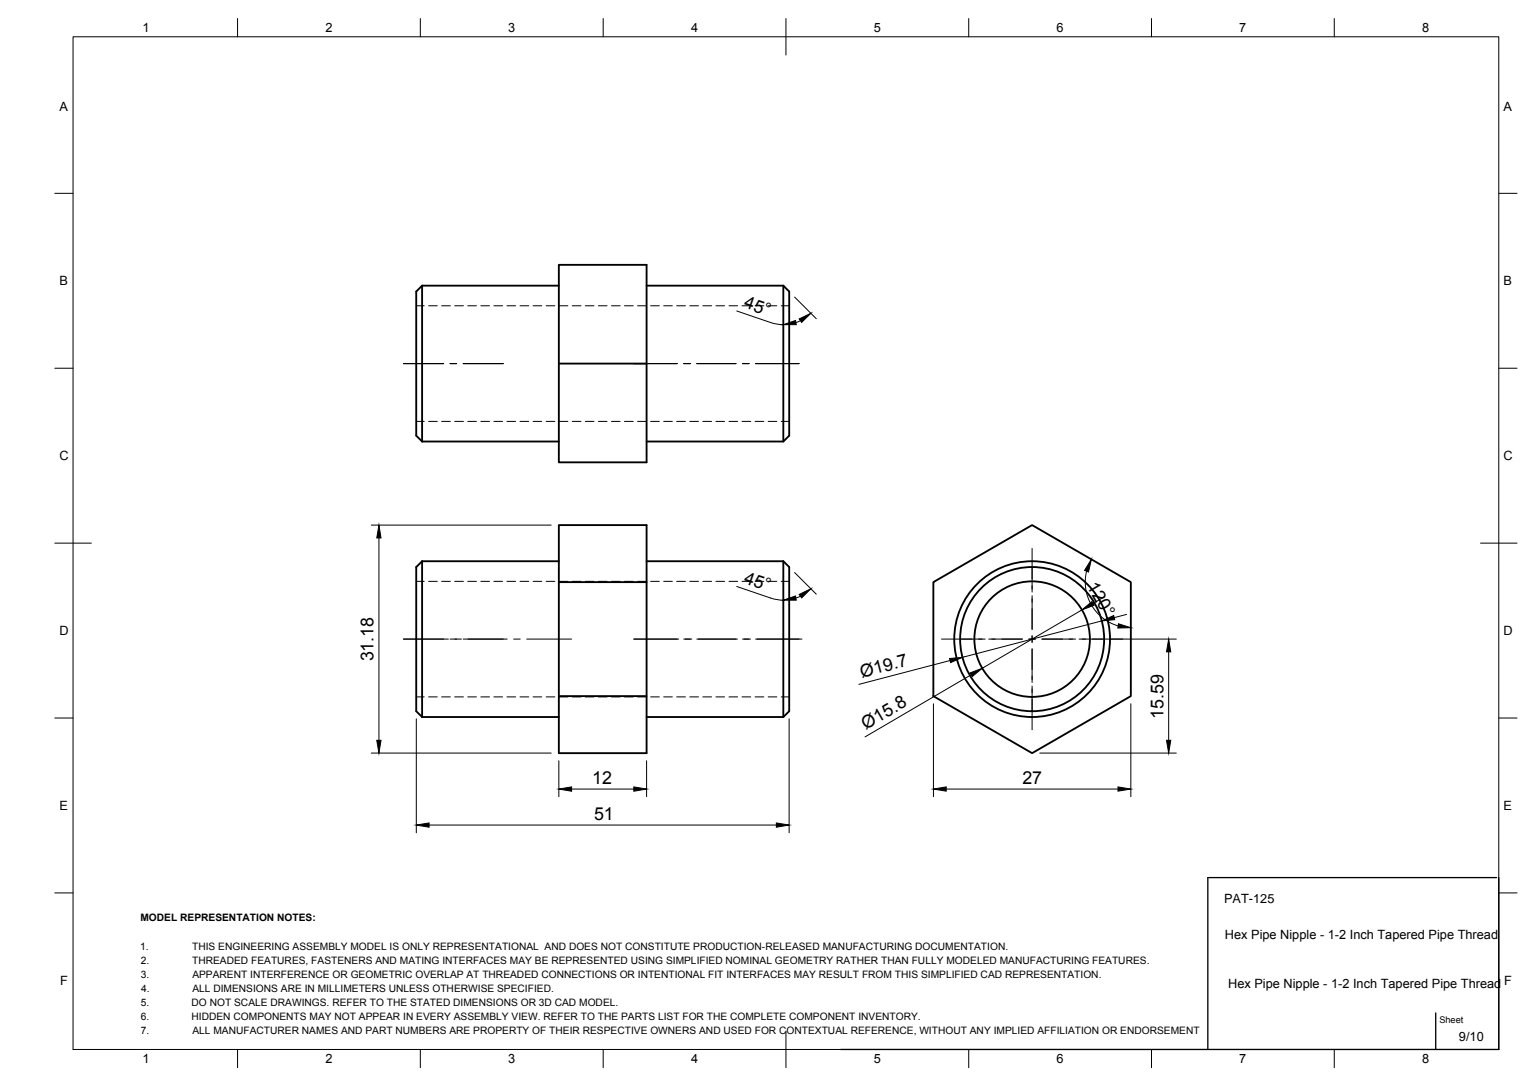
ISO-10303-21;
HEADER;
/* Generated by software containing ST-Developer
 * from STEP Tools, Inc. (www.steptools.com) 
 */

FILE_DESCRIPTION(
/* description */ ('Y-strainer with drain'),
/* implementation_level */ '2;1');

FILE_NAME(
/* name */ 'Hex Pipe Nipple - 1-2 Inch Tapered Pipe Thread.step',
/* time_stamp */ '2026-10-28T00:41:55-07:00',
/* author */ (''),
/* organization */ (''),
/* preprocessor_version */ 'ST-DEVELOPER v20.2',
/* originating_system */ 'Autodesk Translation Framework v15.17.0.0',
/* authorisation */ '');

FILE_SCHEMA (('AUTOMOTIVE_DESIGN { 1 0 10303 214 3 1 1 }'));
ENDSEC;

DATA;
#10=MECHANICAL_DESIGN_GEOMETRIC_PRESENTATION_REPRESENTATION('',(#100),#8864);
#72=CONICAL_SURFACE('',#3736,1.025,0.785398163397448);
#73=CONICAL_SURFACE('',#3739,1.025,0.785398163397448);
#82=SHAPE_REPRESENTATION_RELATIONSHIP('SRR','None',#8914,#91);
#91=ADVANCED_BREP_SHAPE_REPRESENTATION('',(#108),#8862);
#100=STYLED_ITEM('',(#9019),#108);
#108=MANIFOLD_SOLID_BREP('Body1',#3391);
#451=FACE_BOUND('',#932,.T.);
#452=FACE_BOUND('',#934,.T.);
#453=FACE_BOUND('',#943,.T.);
#454=FACE_BOUND('',#948,.T.);
#501=PLANE('',#3721);
#502=PLANE('',#3723);
#503=PLANE('',#3725);
#504=PLANE('',#3726);
#505=PLANE('',#3727);
#506=PLANE('',#3728);
#507=PLANE('',#3729);
#508=PLANE('',#3730);
#509=PLANE('',#3733);
#510=PLANE('',#3741);
#647=FACE_OUTER_BOUND('',#931,.T.);
#648=FACE_OUTER_BOUND('',#933,.T.);
#649=FACE_OUTER_BOUND('',#935,.T.);
#650=FACE_OUTER_BOUND('',#936,.T.);
#651=FACE_OUTER_BOUND('',#937,.T.);
#652=FACE_OUTER_BOUND('',#938,.T.);
#653=FACE_OUTER_BOUND('',#939,.T.);
#654=FACE_OUTER_BOUND('',#940,.T.);
#655=FACE_OUTER_BOUND('',#941,.T.);
#656=FACE_OUTER_BOUND('',#942,.T.);
#657=FACE_OUTER_BOUND('',#944,.T.);
#658=FACE_OUTER_BOUND('',#945,.T.);
#659=FACE_OUTER_BOUND('',#946,.T.);
#660=FACE_OUTER_BOUND('',#947,.T.);
#661=FACE_OUTER_BOUND('',#949,.T.);
#931=EDGE_LOOP('',(#3036,#3037,#3038,#3039,#3040,#3041));
#932=EDGE_LOOP('',(#3042));
#933=EDGE_LOOP('',(#3043,#3044,#3045,#3046,#3047,#3048));
#934=EDGE_LOOP('',(#3049));
#935=EDGE_LOOP('',(#3050,#3051,#3052,#3053));
#936=EDGE_LOOP('',(#3054,#3055,#3056,#3057));
#937=EDGE_LOOP('',(#3058,#3059,#3060,#3061));
#938=EDGE_LOOP('',(#3062,#3063,#3064,#3065));
#939=EDGE_LOOP('',(#3066,#3067,#3068,#3069));
#940=EDGE_LOOP('',(#3070,#3071,#3072,#3073));
#941=EDGE_LOOP('',(#3074,#3075,#3076,#3077));
#942=EDGE_LOOP('',(#3078));
#943=EDGE_LOOP('',(#3079));
#944=EDGE_LOOP('',(#3080,#3081,#3082,#3083));
#945=EDGE_LOOP('',(#3084,#3085,#3086,#3087));
#946=EDGE_LOOP('',(#3088,#3089,#3090,#3091));
#947=EDGE_LOOP('',(#3092));
#948=EDGE_LOOP('',(#3093));
#949=EDGE_LOOP('',(#3094,#3095,#3096,#3097));
#1082=LINE('',#8718,#1245);
#1083=LINE('',#8720,#1246);
#1084=LINE('',#8722,#1247);
#1085=LINE('',#8724,#1248);
#1086=LINE('',#8726,#1249);
#1087=LINE('',#8727,#1250);
#1088=LINE('',#8733,#1251);
#1089=LINE('',#8735,#1252);
#1090=LINE('',#8737,#1253);
#1091=LINE('',#8739,#1254);
#1092=LINE('',#8741,#1255);
#1093=LINE('',#8742,#1256);
#1094=LINE('',#8746,#1257);
#1095=LINE('',#8747,#1258);
#1096=LINE('',#8749,#1259);
#1097=LINE('',#8751,#1260);
#1098=LINE('',#8753,#1261);
#1099=LINE('',#8755,#1262);
#1100=LINE('',#8759,#1263);
#1101=LINE('',#8767,#1264);
#1102=LINE('',#8771,#1265);
#1103=LINE('',#8775,#1266);
#1104=LINE('',#8780,#1267);
#1245=VECTOR('',#4350,1.);
#1246=VECTOR('',#4351,1.);
#1247=VECTOR('',#4352,1.);
#1248=VECTOR('',#4353,1.);
#1249=VECTOR('',#4354,1.);
#1250=VECTOR('',#4355,1.);
#1251=VECTOR('',#4360,1.);
#1252=VECTOR('',#4361,1.);
#1253=VECTOR('',#4362,1.);
#1254=VECTOR('',#4363,1.);
#1255=VECTOR('',#4364,1.);
#1256=VECTOR('',#4365,1.);
#1257=VECTOR('',#4370,1.);
#1258=VECTOR('',#4371,1.);
#1259=VECTOR('',#4374,1.);
#1260=VECTOR('',#4377,1.);
#1261=VECTOR('',#4380,1.);
#1262=VECTOR('',#4383,1.);
#1263=VECTOR('',#4388,1.065);
#1264=VECTOR('',#4399,1.025);
#1265=VECTOR('',#4404,1.065);
#1266=VECTOR('',#4409,1.025);
#1267=VECTOR('',#4416,0.79);
#1369=CIRCLE('',#3722,1.065);
#1370=CIRCLE('',#3724,1.065);
#1371=CIRCLE('',#3732,1.065);
#1372=CIRCLE('',#3734,0.985);
#1373=CIRCLE('',#3735,0.79);
#1374=CIRCLE('',#3738,1.065);
#1375=CIRCLE('',#3740,0.985);
#1376=CIRCLE('',#3742,0.79);
#1687=VERTEX_POINT('',#8716);
#1688=VERTEX_POINT('',#8717);
#1689=VERTEX_POINT('',#8719);
#1690=VERTEX_POINT('',#8721);
#1691=VERTEX_POINT('',#8723);
#1692=VERTEX_POINT('',#8725);
#1693=VERTEX_POINT('',#8728);
#1694=VERTEX_POINT('',#8731);
#1695=VERTEX_POINT('',#8732);
#1696=VERTEX_POINT('',#8734);
#1697=VERTEX_POINT('',#8736);
#1698=VERTEX_POINT('',#8738);
#1699=VERTEX_POINT('',#8740);
#1700=VERTEX_POINT('',#8743);
#1701=VERTEX_POINT('',#8758);
#1702=VERTEX_POINT('',#8762);
#1703=VERTEX_POINT('',#8764);
#1704=VERTEX_POINT('',#8769);
#1705=VERTEX_POINT('',#8773);
#1706=VERTEX_POINT('',#8777);
#2142=EDGE_CURVE('',#1687,#1688,#1082,.T.);
#2143=EDGE_CURVE('',#1688,#1689,#1083,.T.);
#2144=EDGE_CURVE('',#1689,#1690,#1084,.T.);
#2145=EDGE_CURVE('',#1690,#1691,#1085,.T.);
#2146=EDGE_CURVE('',#1691,#1692,#1086,.T.);
#2147=EDGE_CURVE('',#1692,#1687,#1087,.T.);
#2148=EDGE_CURVE('',#1693,#1693,#1369,.T.);
#2149=EDGE_CURVE('',#1694,#1695,#1088,.T.);
#2150=EDGE_CURVE('',#1695,#1696,#1089,.T.);
#2151=EDGE_CURVE('',#1696,#1697,#1090,.T.);
#2152=EDGE_CURVE('',#1697,#1698,#1091,.T.);
#2153=EDGE_CURVE('',#1698,#1699,#1092,.T.);
#2154=EDGE_CURVE('',#1699,#1694,#1093,.T.);
#2155=EDGE_CURVE('',#1700,#1700,#1370,.T.);
#2156=EDGE_CURVE('',#1694,#1688,#1094,.T.);
#2157=EDGE_CURVE('',#1689,#1699,#1095,.T.);
#2158=EDGE_CURVE('',#1690,#1698,#1096,.T.);
#2159=EDGE_CURVE('',#1691,#1697,#1097,.T.);
#2160=EDGE_CURVE('',#1692,#1696,#1098,.T.);
#2161=EDGE_CURVE('',#1687,#1695,#1099,.T.);
#2162=EDGE_CURVE('',#1700,#1701,#1100,.T.);
#2163=EDGE_CURVE('',#1701,#1701,#1371,.T.);
#2164=EDGE_CURVE('',#1702,#1702,#1372,.T.);
#2165=EDGE_CURVE('',#1703,#1703,#1373,.T.);
#2166=EDGE_CURVE('',#1701,#1702,#1101,.T.);
#2167=EDGE_CURVE('',#1704,#1704,#1374,.T.);
#2168=EDGE_CURVE('',#1704,#1693,#1102,.T.);
#2169=EDGE_CURVE('',#1705,#1705,#1375,.T.);
#2170=EDGE_CURVE('',#1705,#1704,#1103,.T.);
#2171=EDGE_CURVE('',#1706,#1706,#1376,.T.);
#2172=EDGE_CURVE('',#1706,#1703,#1104,.T.);
#3036=ORIENTED_EDGE('',*,*,#2142,.T.);
#3037=ORIENTED_EDGE('',*,*,#2143,.T.);
#3038=ORIENTED_EDGE('',*,*,#2144,.T.);
#3039=ORIENTED_EDGE('',*,*,#2145,.T.);
#3040=ORIENTED_EDGE('',*,*,#2146,.T.);
#3041=ORIENTED_EDGE('',*,*,#2147,.T.);
#3042=ORIENTED_EDGE('',*,*,#2148,.F.);
#3043=ORIENTED_EDGE('',*,*,#2149,.T.);
#3044=ORIENTED_EDGE('',*,*,#2150,.T.);
#3045=ORIENTED_EDGE('',*,*,#2151,.T.);
#3046=ORIENTED_EDGE('',*,*,#2152,.T.);
#3047=ORIENTED_EDGE('',*,*,#2153,.T.);
#3048=ORIENTED_EDGE('',*,*,#2154,.T.);
#3049=ORIENTED_EDGE('',*,*,#2155,.F.);
#3050=ORIENTED_EDGE('',*,*,#2156,.F.);
#3051=ORIENTED_EDGE('',*,*,#2154,.F.);
#3052=ORIENTED_EDGE('',*,*,#2157,.F.);
#3053=ORIENTED_EDGE('',*,*,#2143,.F.);
#3054=ORIENTED_EDGE('',*,*,#2157,.T.);
#3055=ORIENTED_EDGE('',*,*,#2153,.F.);
#3056=ORIENTED_EDGE('',*,*,#2158,.F.);
#3057=ORIENTED_EDGE('',*,*,#2144,.F.);
#3058=ORIENTED_EDGE('',*,*,#2158,.T.);
#3059=ORIENTED_EDGE('',*,*,#2152,.F.);
#3060=ORIENTED_EDGE('',*,*,#2159,.F.);
#3061=ORIENTED_EDGE('',*,*,#2145,.F.);
#3062=ORIENTED_EDGE('',*,*,#2159,.T.);
#3063=ORIENTED_EDGE('',*,*,#2151,.F.);
#3064=ORIENTED_EDGE('',*,*,#2160,.F.);
#3065=ORIENTED_EDGE('',*,*,#2146,.F.);
#3066=ORIENTED_EDGE('',*,*,#2160,.T.);
#3067=ORIENTED_EDGE('',*,*,#2150,.F.);
#3068=ORIENTED_EDGE('',*,*,#2161,.F.);
#3069=ORIENTED_EDGE('',*,*,#2147,.F.);
#3070=ORIENTED_EDGE('',*,*,#2161,.T.);
#3071=ORIENTED_EDGE('',*,*,#2149,.F.);
#3072=ORIENTED_EDGE('',*,*,#2156,.T.);
#3073=ORIENTED_EDGE('',*,*,#2142,.F.);
#3074=ORIENTED_EDGE('',*,*,#2155,.T.);
#3075=ORIENTED_EDGE('',*,*,#2162,.T.);
#3076=ORIENTED_EDGE('',*,*,#2163,.T.);
#3077=ORIENTED_EDGE('',*,*,#2162,.F.);
#3078=ORIENTED_EDGE('',*,*,#2164,.F.);
#3079=ORIENTED_EDGE('',*,*,#2165,.T.);
#3080=ORIENTED_EDGE('',*,*,#2163,.F.);
#3081=ORIENTED_EDGE('',*,*,#2166,.T.);
#3082=ORIENTED_EDGE('',*,*,#2164,.T.);
#3083=ORIENTED_EDGE('',*,*,#2166,.F.);
#3084=ORIENTED_EDGE('',*,*,#2167,.F.);
#3085=ORIENTED_EDGE('',*,*,#2168,.T.);
#3086=ORIENTED_EDGE('',*,*,#2148,.T.);
#3087=ORIENTED_EDGE('',*,*,#2168,.F.);
#3088=ORIENTED_EDGE('',*,*,#2169,.F.);
#3089=ORIENTED_EDGE('',*,*,#2170,.T.);
#3090=ORIENTED_EDGE('',*,*,#2167,.T.);
#3091=ORIENTED_EDGE('',*,*,#2170,.F.);
#3092=ORIENTED_EDGE('',*,*,#2169,.T.);
#3093=ORIENTED_EDGE('',*,*,#2171,.F.);
#3094=ORIENTED_EDGE('',*,*,#2171,.T.);
#3095=ORIENTED_EDGE('',*,*,#2172,.T.);
#3096=ORIENTED_EDGE('',*,*,#2165,.F.);
#3097=ORIENTED_EDGE('',*,*,#2172,.F.);
#3227=CYLINDRICAL_SURFACE('',#3731,1.065);
#3228=CYLINDRICAL_SURFACE('',#3737,1.065);
#3229=CYLINDRICAL_SURFACE('',#3743,0.79);
#3358=ADVANCED_FACE('',(#647,#451),#501,.F.);
#3359=ADVANCED_FACE('',(#648,#452),#502,.T.);
#3360=ADVANCED_FACE('',(#649),#503,.T.);
#3361=ADVANCED_FACE('',(#650),#504,.T.);
#3362=ADVANCED_FACE('',(#651),#505,.T.);
#3363=ADVANCED_FACE('',(#652),#506,.T.);
#3364=ADVANCED_FACE('',(#653),#507,.T.);
#3365=ADVANCED_FACE('',(#654),#508,.T.);
#3366=ADVANCED_FACE('',(#655),#3227,.T.);
#3367=ADVANCED_FACE('',(#656,#453),#509,.T.);
#3368=ADVANCED_FACE('',(#657),#72,.T.);
#3369=ADVANCED_FACE('',(#658),#3228,.T.);
#3370=ADVANCED_FACE('',(#659),#73,.T.);
#3371=ADVANCED_FACE('',(#660,#454),#510,.T.);
#3372=ADVANCED_FACE('',(#661),#3229,.F.);
#3391=CLOSED_SHELL('',(#3358,#3359,#3360,#3361,#3362,#3363,#3364,#3365,
#3366,#3367,#3368,#3369,#3370,#3371,#3372));
#3720=AXIS2_PLACEMENT_3D('',#8714,#4346,#4347);
#3721=AXIS2_PLACEMENT_3D('',#8715,#4348,#4349);
#3722=AXIS2_PLACEMENT_3D('',#8729,#4356,#4357);
#3723=AXIS2_PLACEMENT_3D('',#8730,#4358,#4359);
#3724=AXIS2_PLACEMENT_3D('',#8744,#4366,#4367);
#3725=AXIS2_PLACEMENT_3D('',#8745,#4368,#4369);
#3726=AXIS2_PLACEMENT_3D('',#8748,#4372,#4373);
#3727=AXIS2_PLACEMENT_3D('',#8750,#4375,#4376);
#3728=AXIS2_PLACEMENT_3D('',#8752,#4378,#4379);
#3729=AXIS2_PLACEMENT_3D('',#8754,#4381,#4382);
#3730=AXIS2_PLACEMENT_3D('',#8756,#4384,#4385);
#3731=AXIS2_PLACEMENT_3D('',#8757,#4386,#4387);
#3732=AXIS2_PLACEMENT_3D('',#8760,#4389,#4390);
#3733=AXIS2_PLACEMENT_3D('',#8761,#4391,#4392);
#3734=AXIS2_PLACEMENT_3D('',#8763,#4393,#4394);
#3735=AXIS2_PLACEMENT_3D('',#8765,#4395,#4396);
#3736=AXIS2_PLACEMENT_3D('',#8766,#4397,#4398);
#3737=AXIS2_PLACEMENT_3D('',#8768,#4400,#4401);
#3738=AXIS2_PLACEMENT_3D('',#8770,#4402,#4403);
#3739=AXIS2_PLACEMENT_3D('',#8772,#4405,#4406);
#3740=AXIS2_PLACEMENT_3D('',#8774,#4407,#4408);
#3741=AXIS2_PLACEMENT_3D('',#8776,#4410,#4411);
#3742=AXIS2_PLACEMENT_3D('',#8778,#4412,#4413);
#3743=AXIS2_PLACEMENT_3D('',#8779,#4414,#4415);
#4346=DIRECTION('axis',(0.,0.,1.));
#4347=DIRECTION('refdir',(1.,0.,0.));
#4348=DIRECTION('center_axis',(0.,1.,0.));
#4349=DIRECTION('ref_axis',(1.,0.,0.));
#4350=DIRECTION('',(-0.5,0.,0.866025403784439));
#4351=DIRECTION('',(-1.,0.,-2.84883360945713E-16));
#4352=DIRECTION('',(-0.5,0.,-0.866025403784439));
#4353=DIRECTION('',(0.5,0.,-0.866025403784439));
#4354=DIRECTION('',(1.,0.,0.));
#4355=DIRECTION('',(0.5,0.,0.866025403784439));
#4356=DIRECTION('center_axis',(0.,-1.,0.));
#4357=DIRECTION('ref_axis',(1.,0.,0.));
#4358=DIRECTION('center_axis',(0.,1.,0.));
#4359=DIRECTION('ref_axis',(1.,0.,0.));
#4360=DIRECTION('',(0.5,0.,-0.866025403784439));
#4361=DIRECTION('',(-0.5,0.,-0.866025403784439));
#4362=DIRECTION('',(-1.,0.,0.));
#4363=DIRECTION('',(-0.5,0.,0.866025403784439));
#4364=DIRECTION('',(0.5,0.,0.866025403784439));
#4365=DIRECTION('',(1.,0.,2.84883360945713E-16));
#4366=DIRECTION('center_axis',(0.,1.,0.));
#4367=DIRECTION('ref_axis',(1.,0.,0.));
#4368=DIRECTION('center_axis',(-2.84883360945713E-16,0.,1.));
#4369=DIRECTION('ref_axis',(1.,0.,2.84883360945713E-16));
#4370=DIRECTION('',(0.,-1.,0.));
#4371=DIRECTION('',(0.,1.,0.));
#4372=DIRECTION('center_axis',(-0.866025403784439,0.,0.5));
#4373=DIRECTION('ref_axis',(0.5,0.,0.866025403784439));
#4374=DIRECTION('',(0.,1.,0.));
#4375=DIRECTION('center_axis',(-0.866025403784439,0.,-0.5));
#4376=DIRECTION('ref_axis',(-0.5,0.,0.866025403784439));
#4377=DIRECTION('',(0.,1.,0.));
#4378=DIRECTION('center_axis',(0.,0.,-1.));
#4379=DIRECTION('ref_axis',(-1.,0.,0.));
#4380=DIRECTION('',(0.,1.,0.));
#4381=DIRECTION('center_axis',(0.866025403784439,0.,-0.5));
#4382=DIRECTION('ref_axis',(-0.5,0.,-0.866025403784439));
#4383=DIRECTION('',(0.,1.,0.));
#4384=DIRECTION('center_axis',(0.866025403784439,0.,0.5));
#4385=DIRECTION('ref_axis',(0.5,0.,-0.866025403784439));
#4386=DIRECTION('center_axis',(0.,-1.,0.));
#4387=DIRECTION('ref_axis',(1.,0.,0.));
#4388=DIRECTION('',(0.,1.,0.));
#4389=DIRECTION('center_axis',(0.,-1.,0.));
#4390=DIRECTION('ref_axis',(1.,0.,0.));
#4391=DIRECTION('center_axis',(0.,1.,0.));
#4392=DIRECTION('ref_axis',(0.,0.,1.));
#4393=DIRECTION('center_axis',(0.,-1.,0.));
#4394=DIRECTION('ref_axis',(1.,0.,0.));
#4395=DIRECTION('center_axis',(0.,-1.,0.));
#4396=DIRECTION('ref_axis',(1.,0.,0.));
#4397=DIRECTION('center_axis',(0.,-1.,0.));
#4398=DIRECTION('ref_axis',(1.,0.,0.));
#4399=DIRECTION('',(0.707106781186547,0.707106781186548,8.65956056235493E-17));
#4400=DIRECTION('center_axis',(0.,-1.,0.));
#4401=DIRECTION('ref_axis',(1.,0.,0.));
#4402=DIRECTION('center_axis',(0.,-1.,0.));
#4403=DIRECTION('ref_axis',(1.,0.,0.));
#4404=DIRECTION('',(0.,1.,0.));
#4405=DIRECTION('center_axis',(0.,1.,0.));
#4406=DIRECTION('ref_axis',(1.,0.,0.));
#4407=DIRECTION('center_axis',(0.,-1.,0.));
#4408=DIRECTION('ref_axis',(1.,0.,0.));
#4409=DIRECTION('',(-0.707106781186547,0.707106781186548,-8.65956056235493E-17));
#4410=DIRECTION('center_axis',(0.,-1.,0.));
#4411=DIRECTION('ref_axis',(0.,0.,-1.));
#4412=DIRECTION('center_axis',(0.,-1.,0.));
#4413=DIRECTION('ref_axis',(1.,0.,0.));
#4414=DIRECTION('center_axis',(0.,-1.,0.));
#4415=DIRECTION('ref_axis',(1.,0.,0.));
#4416=DIRECTION('',(0.,1.,0.));
#8714=CARTESIAN_POINT('',(0.,0.,0.));
#8715=CARTESIAN_POINT('Origin',(0.,-0.6,0.));
#8716=CARTESIAN_POINT('',(1.55884572681199,-0.6,0.));
#8717=CARTESIAN_POINT('',(0.779422863405995,-0.6,1.35));
#8718=CARTESIAN_POINT('',(0.779422863405995,-0.6,1.35));
#8719=CARTESIAN_POINT('',(-0.779422863405996,-0.6,1.35));
#8720=CARTESIAN_POINT('',(-0.779422863405996,-0.6,1.35));
#8721=CARTESIAN_POINT('',(-1.55884572681199,-0.6,-1.90903542970483E-16));
#8722=CARTESIAN_POINT('',(-1.55884572681199,-0.6,-1.90903542970483E-16));
#8723=CARTESIAN_POINT('',(-0.779422863405995,-0.6,-1.35));
#8724=CARTESIAN_POINT('',(-0.779422863405995,-0.6,-1.35));
#8725=CARTESIAN_POINT('',(0.779422863405995,-0.6,-1.35));
#8726=CARTESIAN_POINT('',(0.779422863405995,-0.6,-1.35));
#8727=CARTESIAN_POINT('',(1.55884572681199,-0.6,0.));
#8728=CARTESIAN_POINT('',(-1.065,-0.6,-1.30424884109193E-16));
#8729=CARTESIAN_POINT('Origin',(0.,-0.6,0.));
#8730=CARTESIAN_POINT('Origin',(0.,0.6,0.));
#8731=CARTESIAN_POINT('',(0.779422863405995,0.6,1.35));
#8732=CARTESIAN_POINT('',(1.55884572681199,0.6,0.));
#8733=CARTESIAN_POINT('',(0.779422863405995,0.6,1.35));
#8734=CARTESIAN_POINT('',(0.779422863405995,0.6,-1.35));
#8735=CARTESIAN_POINT('',(1.55884572681199,0.6,0.));
#8736=CARTESIAN_POINT('',(-0.779422863405995,0.6,-1.35));
#8737=CARTESIAN_POINT('',(0.779422863405995,0.6,-1.35));
#8738=CARTESIAN_POINT('',(-1.55884572681199,0.6,-1.90903542970483E-16));
#8739=CARTESIAN_POINT('',(-0.779422863405995,0.6,-1.35));
#8740=CARTESIAN_POINT('',(-0.779422863405996,0.6,1.35));
#8741=CARTESIAN_POINT('',(-1.55884572681199,0.6,-1.90903542970483E-16));
#8742=CARTESIAN_POINT('',(-0.779422863405996,0.6,1.35));
#8743=CARTESIAN_POINT('',(-1.065,0.6,1.30424884109193E-16));
#8744=CARTESIAN_POINT('Origin',(0.,0.6,0.));
#8745=CARTESIAN_POINT('Origin',(-0.779422863405996,0.,1.35));
#8746=CARTESIAN_POINT('',(0.779422863405995,0.,1.35));
#8747=CARTESIAN_POINT('',(-0.779422863405996,0.,1.35));
#8748=CARTESIAN_POINT('Origin',(-1.55884572681199,0.,-1.90903542970483E-16));
#8749=CARTESIAN_POINT('',(-1.55884572681199,0.,-1.90903542970483E-16));
#8750=CARTESIAN_POINT('Origin',(-0.779422863405995,0.,-1.35));
#8751=CARTESIAN_POINT('',(-0.779422863405995,0.,-1.35));
#8752=CARTESIAN_POINT('Origin',(0.779422863405995,0.,-1.35));
#8753=CARTESIAN_POINT('',(0.779422863405995,0.,-1.35));
#8754=CARTESIAN_POINT('Origin',(1.55884572681199,0.,0.));
#8755=CARTESIAN_POINT('',(1.55884572681199,0.,0.));
#8756=CARTESIAN_POINT('Origin',(0.779422863405995,0.,1.35));
#8757=CARTESIAN_POINT('Origin',(0.,0.,0.));
#8758=CARTESIAN_POINT('',(-1.065,2.47,-1.30424884109193E-16));
#8759=CARTESIAN_POINT('',(-1.065,0.,-1.30424884109193E-16));
#8760=CARTESIAN_POINT('Origin',(0.,2.47,0.));
#8761=CARTESIAN_POINT('Origin',(0.985,2.55,0.));
#8762=CARTESIAN_POINT('',(-0.985,2.55,-1.20627709716014E-16));
#8763=CARTESIAN_POINT('Origin',(0.,2.55,0.));
#8764=CARTESIAN_POINT('',(-0.79,2.55,-9.67470971326409E-17));
#8765=CARTESIAN_POINT('Origin',(0.,2.55,0.));
#8766=CARTESIAN_POINT('Origin',(0.,2.51,0.));
#8767=CARTESIAN_POINT('',(-1.025,2.51,-1.25526296912604E-16));
#8768=CARTESIAN_POINT('Origin',(0.,0.,0.));
#8769=CARTESIAN_POINT('',(-1.065,-2.47,-1.30424884109193E-16));
#8770=CARTESIAN_POINT('Origin',(0.,-2.47,0.));
#8771=CARTESIAN_POINT('',(-1.065,0.,-1.30424884109193E-16));
#8772=CARTESIAN_POINT('Origin',(0.,-2.51,0.));
#8773=CARTESIAN_POINT('',(-0.985,-2.55,-1.20627709716014E-16));
#8774=CARTESIAN_POINT('Origin',(0.,-2.55,0.));
#8775=CARTESIAN_POINT('',(-1.025,-2.51,-1.25526296912604E-16));
#8776=CARTESIAN_POINT('Origin',(0.79,-2.55,0.));
#8777=CARTESIAN_POINT('',(-0.79,-2.55,-9.67470971326409E-17));
#8778=CARTESIAN_POINT('Origin',(0.,-2.55,0.));
#8779=CARTESIAN_POINT('Origin',(0.,0.,0.));
#8780=CARTESIAN_POINT('',(-0.79,0.,-9.67470971326409E-17));
#8850=UNCERTAINTY_MEASURE_WITH_UNIT(LENGTH_MEASURE(0.001),#8865,
'DISTANCE_ACCURACY_VALUE',
'Maximum model space distance between geometric entities at asserted c
onnectivities');
#8852=UNCERTAINTY_MEASURE_WITH_UNIT(LENGTH_MEASURE(0.001),#8865,
'DISTANCE_ACCURACY_VALUE',
'Maximum model space distance between geometric entities at asserted c
onnectivities');
#8862=(
GEOMETRIC_REPRESENTATION_CONTEXT(3)
GLOBAL_UNCERTAINTY_ASSIGNED_CONTEXT((#8850))
GLOBAL_UNIT_ASSIGNED_CONTEXT((#8865,#8867,#8868))
REPRESENTATION_CONTEXT('','3D')
);
#8864=(
GEOMETRIC_REPRESENTATION_CONTEXT(3)
GLOBAL_UNCERTAINTY_ASSIGNED_CONTEXT((#8852))
GLOBAL_UNIT_ASSIGNED_CONTEXT((#8865,#8867,#8868))
REPRESENTATION_CONTEXT('','3D')
);
#8865=(
LENGTH_UNIT()
NAMED_UNIT(*)
SI_UNIT(.CENTI.,.METRE.)
);
#8867=(
NAMED_UNIT(*)
PLANE_ANGLE_UNIT()
SI_UNIT($,.RADIAN.)
);
#8868=(
NAMED_UNIT(*)
SI_UNIT($,.STERADIAN.)
SOLID_ANGLE_UNIT()
);
#8878=SHAPE_DEFINITION_REPRESENTATION(#8889,#8914);
#8889=PRODUCT_DEFINITION_SHAPE('',$,#8926);
#8914=SHAPE_REPRESENTATION('',(#3720),#8862);
#8916=PRODUCT_DEFINITION_CONTEXT('part definition',#8951,'design');
#8926=PRODUCT_DEFINITION(
'Hex Pipe Nipple - 1-2 Inch Tapered Pipe Thread',
'Hex Pipe Nipple - 1-2 Inch Tapered Pipe Thread',#8937,#8916);
#8937=PRODUCT_DEFINITION_FORMATION('',$,#8962);
#8951=APPLICATION_CONTEXT(
'Core Data for Automotive Mechanical Design Process');
#8952=PRODUCT_CONTEXT('part definition',#8951,'mechanical');
#8962=PRODUCT('Hex Pipe Nipple - 1-2 Inch Tapered Pipe Thread',
'Hex Pipe Nipple - 1-2 Inch Tapered Pipe Thread',
'Hex Pipe Nipple - 1-2 Inch Tapered Pipe Thread',(#8952));
#9013=COLOUR_RGB('Light Blue',0.38,0.62,0.78);
#9014=FILL_AREA_STYLE_COLOUR('',#9013);
#9015=FILL_AREA_STYLE('',(#9014));
#9016=SURFACE_STYLE_FILL_AREA(#9015);
#9017=SURFACE_SIDE_STYLE('',(#9016));
#9018=SURFACE_STYLE_USAGE(.BOTH.,#9017);
#9019=PRESENTATION_STYLE_ASSIGNMENT((#9018));
ENDSEC;
END-ISO-10303-21;
